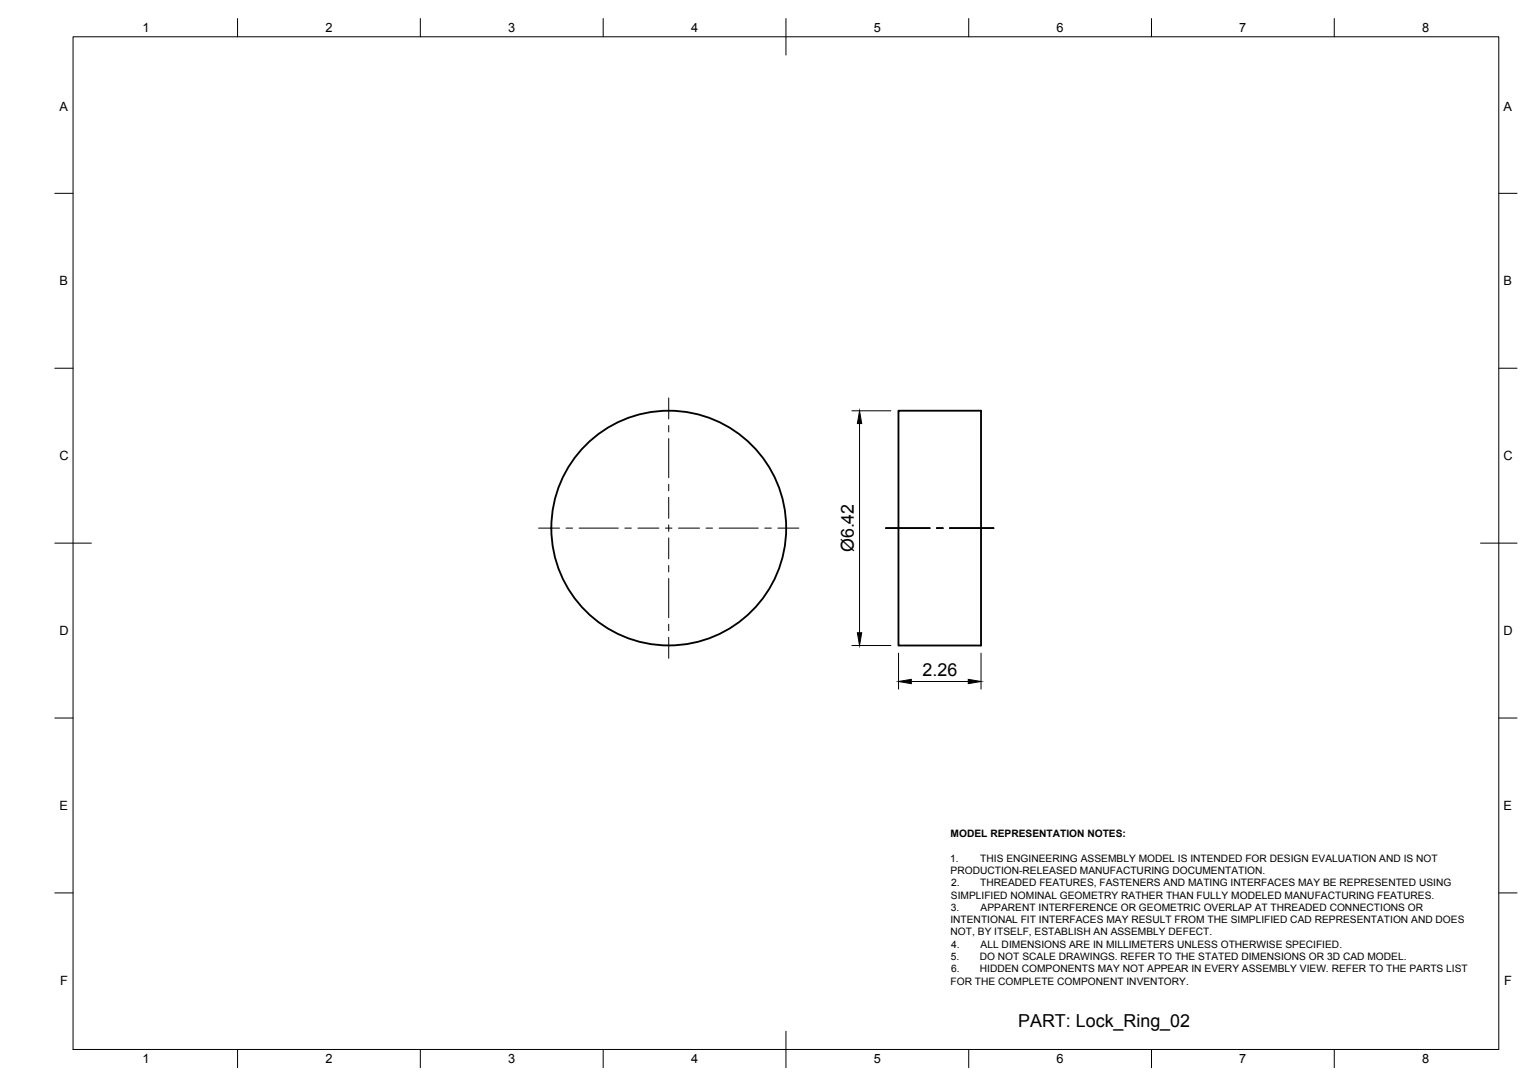
ISO-10303-21;
HEADER;
/* Generated by software containing ST-Developer
 * from STEP Tools, Inc. (www.steptools.com) 
 */

FILE_DESCRIPTION(
/* description */ (''),
/* implementation_level */ '2;1');

FILE_NAME(
/* name */ 'Lock_Ring_02.step',
/* time_stamp */ '2026-10-05T01:33:24-07:00',
/* author */ (''),
/* organization */ (''),
/* preprocessor_version */ 'ST-DEVELOPER v20.2',
/* originating_system */ 'Autodesk Translation Framework v15.15.0.0',
/* authorisation */ '');

FILE_SCHEMA (('AUTOMOTIVE_DESIGN { 1 0 10303 214 3 1 1 }'));
ENDSEC;

DATA;
#10=MECHANICAL_DESIGN_GEOMETRIC_PRESENTATION_REPRESENTATION('',(#84),#1128);
#64=SHAPE_REPRESENTATION_RELATIONSHIP('SRR','None',#1168,#74);
#74=ADVANCED_BREP_SHAPE_REPRESENTATION('',(#94),#1120);
#84=STYLED_ITEM('',(#1226),#94);
#94=MANIFOLD_SOLID_BREP('Body1',#523);
#107=LINE('',#996,#124);
#124=VECTOR('',#796,3.21047290937838);
#139=CYLINDRICAL_SURFACE('',#665,3.21047290937838);
#156=FACE_OUTER_BOUND('',#197,.T.);
#157=FACE_OUTER_BOUND('',#198,.T.);
#158=FACE_OUTER_BOUND('',#199,.T.);
#197=EDGE_LOOP('',(#380,#381,#382,#383));
#198=EDGE_LOOP('',(#384));
#199=EDGE_LOOP('',(#385));
#237=CIRCLE('',#666,3.21047290937838);
#238=CIRCLE('',#667,3.21047290937838);
#273=VERTEX_POINT('',#993);
#274=VERTEX_POINT('',#995);
#312=EDGE_CURVE('',#273,#273,#237,.T.);
#313=EDGE_CURVE('',#273,#274,#107,.T.);
#314=EDGE_CURVE('',#274,#274,#238,.T.);
#380=ORIENTED_EDGE('',*,*,#312,.F.);
#381=ORIENTED_EDGE('',*,*,#313,.T.);
#382=ORIENTED_EDGE('',*,*,#314,.T.);
#383=ORIENTED_EDGE('',*,*,#313,.F.);
#384=ORIENTED_EDGE('',*,*,#312,.T.);
#385=ORIENTED_EDGE('',*,*,#314,.F.);
#464=PLANE('',#668);
#465=PLANE('',#669);
#490=ADVANCED_FACE('',(#156),#139,.T.);
#491=ADVANCED_FACE('',(#157),#464,.T.);
#492=ADVANCED_FACE('',(#158),#465,.T.);
#523=CLOSED_SHELL('',(#490,#491,#492));
#664=AXIS2_PLACEMENT_3D('',#991,#790,#791);
#665=AXIS2_PLACEMENT_3D('',#992,#792,#793);
#666=AXIS2_PLACEMENT_3D('',#994,#794,#795);
#667=AXIS2_PLACEMENT_3D('',#997,#797,#798);
#668=AXIS2_PLACEMENT_3D('',#998,#799,#800);
#669=AXIS2_PLACEMENT_3D('',#999,#801,#802);
#790=DIRECTION('axis',(0.,0.,1.));
#791=DIRECTION('refdir',(1.,0.,0.));
#792=DIRECTION('center_axis',(1.,0.,0.));
#793=DIRECTION('ref_axis',(0.,0.,-1.));
#794=DIRECTION('center_axis',(1.,0.,0.));
#795=DIRECTION('ref_axis',(0.,0.,-1.));
#796=DIRECTION('',(-1.,0.,0.));
#797=DIRECTION('center_axis',(1.,0.,0.));
#798=DIRECTION('ref_axis',(0.,0.,-1.));
#799=DIRECTION('center_axis',(1.,0.,0.));
#800=DIRECTION('ref_axis',(0.,0.,-1.));
#801=DIRECTION('center_axis',(-1.,0.,0.));
#802=DIRECTION('ref_axis',(0.,0.,1.));
#991=CARTESIAN_POINT('',(0.,0.,0.));
#992=CARTESIAN_POINT('Origin',(87.7281259529897,0.,0.));
#993=CARTESIAN_POINT('',(88.8564620398316,-3.93169537221952E-16,3.21047290937838));
#994=CARTESIAN_POINT('Origin',(88.8564620398316,0.,0.));
#995=CARTESIAN_POINT('',(86.5997898661478,-3.93169537221952E-16,3.21047290937838));
#996=CARTESIAN_POINT('',(87.7281259529897,-3.93169537221952E-16,3.21047290937838));
#997=CARTESIAN_POINT('Origin',(86.5997898661478,0.,0.));
#998=CARTESIAN_POINT('Origin',(88.8564620398316,0.,0.));
#999=CARTESIAN_POINT('Origin',(86.5997898661478,0.,-3.21047290937838));
#1108=UNCERTAINTY_MEASURE_WITH_UNIT(LENGTH_MEASURE(0.01),#1129,
'DISTANCE_ACCURACY_VALUE',
'Maximum model space distance between geometric entities at asserted c
onnectivities');
#1116=UNCERTAINTY_MEASURE_WITH_UNIT(LENGTH_MEASURE(0.01),#1129,
'DISTANCE_ACCURACY_VALUE',
'Maximum model space distance between geometric entities at asserted c
onnectivities');
#1120=(
GEOMETRIC_REPRESENTATION_CONTEXT(3)
GLOBAL_UNCERTAINTY_ASSIGNED_CONTEXT((#1108))
GLOBAL_UNIT_ASSIGNED_CONTEXT((#1129,#1131,#1132))
REPRESENTATION_CONTEXT('','3D')
);
#1128=(
GEOMETRIC_REPRESENTATION_CONTEXT(3)
GLOBAL_UNCERTAINTY_ASSIGNED_CONTEXT((#1116))
GLOBAL_UNIT_ASSIGNED_CONTEXT((#1129,#1131,#1132))
REPRESENTATION_CONTEXT('','3D')
);
#1129=(
LENGTH_UNIT()
NAMED_UNIT(*)
SI_UNIT(.MILLI.,.METRE.)
);
#1131=(
NAMED_UNIT(*)
PLANE_ANGLE_UNIT()
SI_UNIT($,.RADIAN.)
);
#1132=(
NAMED_UNIT(*)
SI_UNIT($,.STERADIAN.)
SOLID_ANGLE_UNIT()
);
#1136=SHAPE_DEFINITION_REPRESENTATION(#1147,#1168);
#1147=PRODUCT_DEFINITION_SHAPE('',$,#1180);
#1168=SHAPE_REPRESENTATION('',(#664),#1120);
#1176=PRODUCT_DEFINITION_CONTEXT('part definition',#1211,'design');
#1180=PRODUCT_DEFINITION('Lock_Ring_02','Lock_Ring_02',#1191,#1176);
#1191=PRODUCT_DEFINITION_FORMATION('',$,#1216);
#1211=APPLICATION_CONTEXT(
'Core Data for Automotive Mechanical Design Process');
#1212=PRODUCT_CONTEXT('part definition',#1211,'mechanical');
#1216=PRODUCT('Lock_Ring_02','Lock_Ring_02',$,(#1212));
#1226=PRESENTATION_STYLE_ASSIGNMENT((#1230));
#1230=SURFACE_STYLE_USAGE(.BOTH.,#1234);
#1234=SURFACE_SIDE_STYLE('',(#1238));
#1238=SURFACE_STYLE_FILL_AREA(#1242);
#1242=FILL_AREA_STYLE('Opaque(94,95,15)',(#1246));
#1246=FILL_AREA_STYLE_COLOUR('Opaque(94,95,15)',#1250);
#1250=COLOUR_RGB('Opaque(94,95,15)', 0.31764706, 0.68627451, 0.89019608);
ENDSEC;
END-ISO-10303-21;
